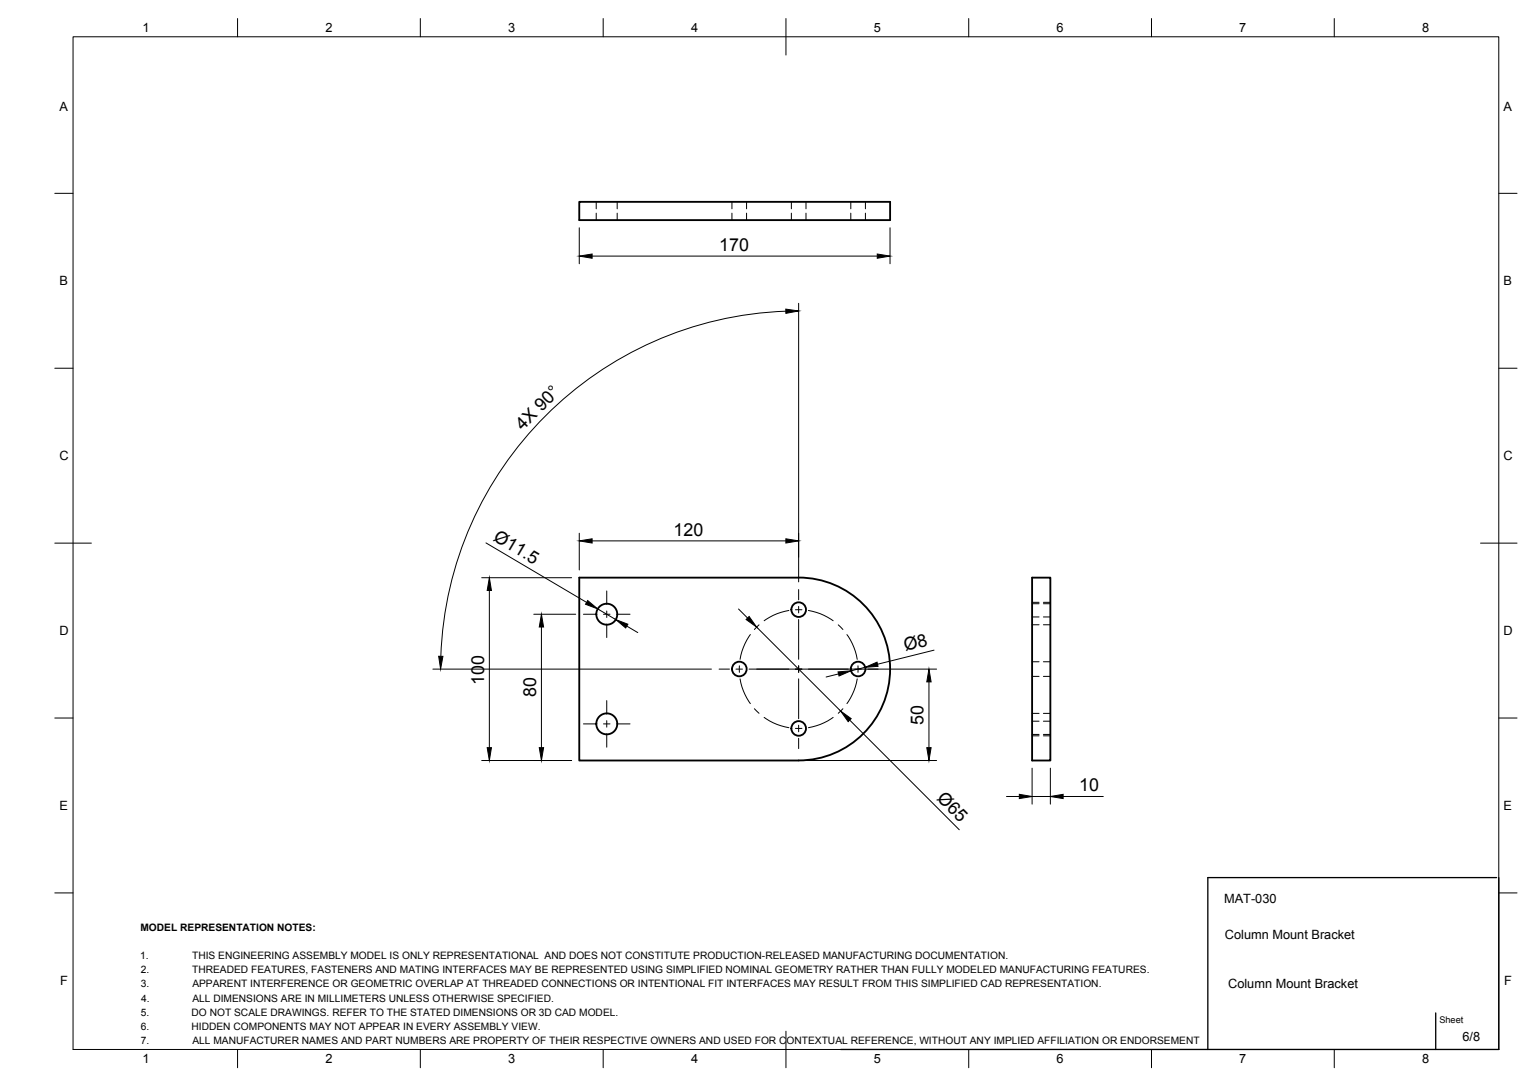
ISO-10303-21;
HEADER;
/* Generated by software containing ST-Developer
 * from STEP Tools, Inc. (www.steptools.com) 
 */

FILE_DESCRIPTION(
/* description */ ('STEP AP214'),
/* implementation_level */ '2;1');

FILE_NAME(
/* name */ 'Column Mount Bracket.step',
/* time_stamp */ '2026-11-14T06:43:04-08:00',
/* author */ (''),
/* organization */ (''),
/* preprocessor_version */ 'ST-DEVELOPER v20.2',
/* originating_system */ 'Autodesk Translation Framework v15.17.0.0',
/* authorisation */ '');

FILE_SCHEMA (('AUTOMOTIVE_DESIGN { 1 0 10303 214 3 1 1 }'));
ENDSEC;

DATA;
#10=MECHANICAL_DESIGN_GEOMETRIC_PRESENTATION_REPRESENTATION('',(#199),#5658);
#177=SHAPE_REPRESENTATION_RELATIONSHIP('SRR','None',#5707,#188);
#188=ADVANCED_BREP_SHAPE_REPRESENTATION('',(#210),#5648);
#199=STYLED_ITEM('',(#5771),#210);
#210=MANIFOLD_SOLID_BREP('Body1',#3061);
#224=CYLINDRICAL_SURFACE('',#3214,4.);
#225=CYLINDRICAL_SURFACE('',#3217,4.);
#226=CYLINDRICAL_SURFACE('',#3220,4.);
#227=CYLINDRICAL_SURFACE('',#3223,3.99999999999999);
#228=CYLINDRICAL_SURFACE('',#3226,5.75);
#229=CYLINDRICAL_SURFACE('',#3229,5.75000000000001);
#230=CYLINDRICAL_SURFACE('',#3238,50.0000000000001);
#273=FACE_BOUND('',#538,.T.);
#274=FACE_BOUND('',#539,.T.);
#275=FACE_BOUND('',#540,.T.);
#276=FACE_BOUND('',#541,.T.);
#277=FACE_BOUND('',#542,.T.);
#278=FACE_BOUND('',#543,.T.);
#279=FACE_BOUND('',#545,.T.);
#280=FACE_BOUND('',#546,.T.);
#281=FACE_BOUND('',#547,.T.);
#282=FACE_BOUND('',#548,.T.);
#283=FACE_BOUND('',#549,.T.);
#284=FACE_BOUND('',#550,.T.);
#347=FACE_OUTER_BOUND('',#531,.T.);
#348=FACE_OUTER_BOUND('',#532,.T.);
#349=FACE_OUTER_BOUND('',#533,.T.);
#350=FACE_OUTER_BOUND('',#534,.T.);
#351=FACE_OUTER_BOUND('',#535,.T.);
#352=FACE_OUTER_BOUND('',#536,.T.);
#353=FACE_OUTER_BOUND('',#537,.T.);
#354=FACE_OUTER_BOUND('',#544,.T.);
#355=FACE_OUTER_BOUND('',#551,.T.);
#356=FACE_OUTER_BOUND('',#552,.T.);
#357=FACE_OUTER_BOUND('',#553,.T.);
#358=FACE_OUTER_BOUND('',#554,.T.);
#531=EDGE_LOOP('',(#2024,#2025,#2026,#2027));
#532=EDGE_LOOP('',(#2028,#2029,#2030,#2031));
#533=EDGE_LOOP('',(#2032,#2033,#2034,#2035));
#534=EDGE_LOOP('',(#2036,#2037,#2038,#2039));
#535=EDGE_LOOP('',(#2040,#2041,#2042,#2043));
#536=EDGE_LOOP('',(#2044,#2045,#2046,#2047));
#537=EDGE_LOOP('',(#2048,#2049,#2050,#2051));
#538=EDGE_LOOP('',(#2052));
#539=EDGE_LOOP('',(#2053));
#540=EDGE_LOOP('',(#2054));
#541=EDGE_LOOP('',(#2055));
#542=EDGE_LOOP('',(#2056));
#543=EDGE_LOOP('',(#2057));
#544=EDGE_LOOP('',(#2058,#2059,#2060,#2061));
#545=EDGE_LOOP('',(#2062));
#546=EDGE_LOOP('',(#2063));
#547=EDGE_LOOP('',(#2064));
#548=EDGE_LOOP('',(#2065));
#549=EDGE_LOOP('',(#2066));
#550=EDGE_LOOP('',(#2067));
#551=EDGE_LOOP('',(#2068,#2069,#2070,#2071));
#552=EDGE_LOOP('',(#2072,#2073,#2074,#2075));
#553=EDGE_LOOP('',(#2076,#2077,#2078,#2079));
#554=EDGE_LOOP('',(#2080,#2081,#2082,#2083));
#783=LINE('',#4544,#979);
#784=LINE('',#4550,#980);
#785=LINE('',#4556,#981);
#786=LINE('',#4562,#982);
#787=LINE('',#4568,#983);
#788=LINE('',#4574,#984);
#789=LINE('',#4579,#985);
#790=LINE('',#4581,#986);
#791=LINE('',#4584,#987);
#792=LINE('',#4588,#988);
#793=LINE('',#4590,#989);
#794=LINE('',#4593,#990);
#795=LINE('',#4595,#991);
#796=LINE('',#4596,#992);
#797=LINE('',#4598,#993);
#798=LINE('',#4600,#994);
#979=VECTOR('',#3621,4.);
#980=VECTOR('',#3628,4.);
#981=VECTOR('',#3635,4.);
#982=VECTOR('',#3642,3.99999999999999);
#983=VECTOR('',#3649,5.75);
#984=VECTOR('',#3656,5.75000000000001);
#985=VECTOR('',#3661,1000.);
#986=VECTOR('',#3662,1000.);
#987=VECTOR('',#3665,1000.);
#988=VECTOR('',#3668,1000.);
#989=VECTOR('',#3669,1000.);
#990=VECTOR('',#3672,1000.);
#991=VECTOR('',#3675,1000.);
#992=VECTOR('',#3676,1000.);
#993=VECTOR('',#3679,1000.);
#994=VECTOR('',#3682,1000.);
#1167=CIRCLE('',#3215,4.);
#1168=CIRCLE('',#3216,4.);
#1169=CIRCLE('',#3218,4.);
#1170=CIRCLE('',#3219,4.);
#1171=CIRCLE('',#3221,4.00000000000001);
#1172=CIRCLE('',#3222,4.00000000000001);
#1173=CIRCLE('',#3224,3.99999999999999);
#1174=CIRCLE('',#3225,3.99999999999999);
#1175=CIRCLE('',#3227,5.75);
#1176=CIRCLE('',#3228,5.75);
#1177=CIRCLE('',#3230,5.75000000000001);
#1178=CIRCLE('',#3231,5.75000000000001);
#1179=CIRCLE('',#3233,50.0000000000001);
#1180=CIRCLE('',#3235,50.0000000000001);
#1330=VERTEX_POINT('',#4541);
#1331=VERTEX_POINT('',#4543);
#1332=VERTEX_POINT('',#4547);
#1333=VERTEX_POINT('',#4549);
#1334=VERTEX_POINT('',#4553);
#1335=VERTEX_POINT('',#4555);
#1336=VERTEX_POINT('',#4559);
#1337=VERTEX_POINT('',#4561);
#1338=VERTEX_POINT('',#4565);
#1339=VERTEX_POINT('',#4567);
#1340=VERTEX_POINT('',#4571);
#1341=VERTEX_POINT('',#4573);
#1342=VERTEX_POINT('',#4577);
#1343=VERTEX_POINT('',#4578);
#1344=VERTEX_POINT('',#4580);
#1345=VERTEX_POINT('',#4582);
#1346=VERTEX_POINT('',#4586);
#1347=VERTEX_POINT('',#4587);
#1348=VERTEX_POINT('',#4589);
#1349=VERTEX_POINT('',#4591);
#1595=EDGE_CURVE('',#1330,#1330,#1167,.T.);
#1596=EDGE_CURVE('',#1330,#1331,#783,.T.);
#1597=EDGE_CURVE('',#1331,#1331,#1168,.T.);
#1598=EDGE_CURVE('',#1332,#1332,#1169,.T.);
#1599=EDGE_CURVE('',#1332,#1333,#784,.T.);
#1600=EDGE_CURVE('',#1333,#1333,#1170,.T.);
#1601=EDGE_CURVE('',#1334,#1334,#1171,.T.);
#1602=EDGE_CURVE('',#1334,#1335,#785,.T.);
#1603=EDGE_CURVE('',#1335,#1335,#1172,.T.);
#1604=EDGE_CURVE('',#1336,#1336,#1173,.T.);
#1605=EDGE_CURVE('',#1336,#1337,#786,.T.);
#1606=EDGE_CURVE('',#1337,#1337,#1174,.T.);
#1607=EDGE_CURVE('',#1338,#1338,#1175,.T.);
#1608=EDGE_CURVE('',#1338,#1339,#787,.T.);
#1609=EDGE_CURVE('',#1339,#1339,#1176,.T.);
#1610=EDGE_CURVE('',#1340,#1340,#1177,.T.);
#1611=EDGE_CURVE('',#1340,#1341,#788,.T.);
#1612=EDGE_CURVE('',#1341,#1341,#1178,.T.);
#1613=EDGE_CURVE('',#1342,#1343,#789,.T.);
#1614=EDGE_CURVE('',#1343,#1344,#790,.T.);
#1615=EDGE_CURVE('',#1344,#1345,#1179,.T.);
#1616=EDGE_CURVE('',#1345,#1342,#791,.T.);
#1617=EDGE_CURVE('',#1346,#1347,#792,.T.);
#1618=EDGE_CURVE('',#1348,#1346,#793,.T.);
#1619=EDGE_CURVE('',#1349,#1348,#1180,.T.);
#1620=EDGE_CURVE('',#1347,#1349,#794,.T.);
#1621=EDGE_CURVE('',#1343,#1347,#795,.T.);
#1622=EDGE_CURVE('',#1342,#1346,#796,.T.);
#1623=EDGE_CURVE('',#1344,#1349,#797,.T.);
#1624=EDGE_CURVE('',#1345,#1348,#798,.T.);
#2024=ORIENTED_EDGE('',*,*,#1595,.T.);
#2025=ORIENTED_EDGE('',*,*,#1596,.T.);
#2026=ORIENTED_EDGE('',*,*,#1597,.F.);
#2027=ORIENTED_EDGE('',*,*,#1596,.F.);
#2028=ORIENTED_EDGE('',*,*,#1598,.T.);
#2029=ORIENTED_EDGE('',*,*,#1599,.T.);
#2030=ORIENTED_EDGE('',*,*,#1600,.F.);
#2031=ORIENTED_EDGE('',*,*,#1599,.F.);
#2032=ORIENTED_EDGE('',*,*,#1601,.T.);
#2033=ORIENTED_EDGE('',*,*,#1602,.T.);
#2034=ORIENTED_EDGE('',*,*,#1603,.F.);
#2035=ORIENTED_EDGE('',*,*,#1602,.F.);
#2036=ORIENTED_EDGE('',*,*,#1604,.T.);
#2037=ORIENTED_EDGE('',*,*,#1605,.T.);
#2038=ORIENTED_EDGE('',*,*,#1606,.F.);
#2039=ORIENTED_EDGE('',*,*,#1605,.F.);
#2040=ORIENTED_EDGE('',*,*,#1607,.T.);
#2041=ORIENTED_EDGE('',*,*,#1608,.T.);
#2042=ORIENTED_EDGE('',*,*,#1609,.F.);
#2043=ORIENTED_EDGE('',*,*,#1608,.F.);
#2044=ORIENTED_EDGE('',*,*,#1610,.T.);
#2045=ORIENTED_EDGE('',*,*,#1611,.T.);
#2046=ORIENTED_EDGE('',*,*,#1612,.F.);
#2047=ORIENTED_EDGE('',*,*,#1611,.F.);
#2048=ORIENTED_EDGE('',*,*,#1613,.T.);
#2049=ORIENTED_EDGE('',*,*,#1614,.T.);
#2050=ORIENTED_EDGE('',*,*,#1615,.T.);
#2051=ORIENTED_EDGE('',*,*,#1616,.T.);
#2052=ORIENTED_EDGE('',*,*,#1607,.F.);
#2053=ORIENTED_EDGE('',*,*,#1601,.F.);
#2054=ORIENTED_EDGE('',*,*,#1595,.F.);
#2055=ORIENTED_EDGE('',*,*,#1598,.F.);
#2056=ORIENTED_EDGE('',*,*,#1604,.F.);
#2057=ORIENTED_EDGE('',*,*,#1610,.F.);
#2058=ORIENTED_EDGE('',*,*,#1617,.F.);
#2059=ORIENTED_EDGE('',*,*,#1618,.F.);
#2060=ORIENTED_EDGE('',*,*,#1619,.F.);
#2061=ORIENTED_EDGE('',*,*,#1620,.F.);
#2062=ORIENTED_EDGE('',*,*,#1612,.T.);
#2063=ORIENTED_EDGE('',*,*,#1609,.T.);
#2064=ORIENTED_EDGE('',*,*,#1606,.T.);
#2065=ORIENTED_EDGE('',*,*,#1603,.T.);
#2066=ORIENTED_EDGE('',*,*,#1600,.T.);
#2067=ORIENTED_EDGE('',*,*,#1597,.T.);
#2068=ORIENTED_EDGE('',*,*,#1617,.T.);
#2069=ORIENTED_EDGE('',*,*,#1621,.F.);
#2070=ORIENTED_EDGE('',*,*,#1613,.F.);
#2071=ORIENTED_EDGE('',*,*,#1622,.T.);
#2072=ORIENTED_EDGE('',*,*,#1620,.T.);
#2073=ORIENTED_EDGE('',*,*,#1623,.F.);
#2074=ORIENTED_EDGE('',*,*,#1614,.F.);
#2075=ORIENTED_EDGE('',*,*,#1621,.T.);
#2076=ORIENTED_EDGE('',*,*,#1619,.T.);
#2077=ORIENTED_EDGE('',*,*,#1624,.F.);
#2078=ORIENTED_EDGE('',*,*,#1615,.F.);
#2079=ORIENTED_EDGE('',*,*,#1623,.T.);
#2080=ORIENTED_EDGE('',*,*,#1618,.T.);
#2081=ORIENTED_EDGE('',*,*,#1622,.F.);
#2082=ORIENTED_EDGE('',*,*,#1616,.F.);
#2083=ORIENTED_EDGE('',*,*,#1624,.T.);
#2792=PLANE('',#3232);
#2793=PLANE('',#3234);
#2794=PLANE('',#3236);
#2795=PLANE('',#3237);
#2796=PLANE('',#3239);
#2888=ADVANCED_FACE('',(#347),#224,.F.);
#2889=ADVANCED_FACE('',(#348),#225,.F.);
#2890=ADVANCED_FACE('',(#349),#226,.F.);
#2891=ADVANCED_FACE('',(#350),#227,.F.);
#2892=ADVANCED_FACE('',(#351),#228,.F.);
#2893=ADVANCED_FACE('',(#352),#229,.F.);
#2894=ADVANCED_FACE('',(#353,#273,#274,#275,#276,#277,#278),#2792,.T.);
#2895=ADVANCED_FACE('',(#354,#279,#280,#281,#282,#283,#284),#2793,.F.);
#2896=ADVANCED_FACE('',(#355),#2794,.F.);
#2897=ADVANCED_FACE('',(#356),#2795,.F.);
#2898=ADVANCED_FACE('',(#357),#230,.T.);
#2899=ADVANCED_FACE('',(#358),#2796,.F.);
#3061=CLOSED_SHELL('',(#2888,#2889,#2890,#2891,#2892,#2893,#2894,#2895,
#2896,#2897,#2898,#2899));
#3213=AXIS2_PLACEMENT_3D('',#4539,#3615,#3616);
#3214=AXIS2_PLACEMENT_3D('',#4540,#3617,#3618);
#3215=AXIS2_PLACEMENT_3D('',#4542,#3619,#3620);
#3216=AXIS2_PLACEMENT_3D('',#4545,#3622,#3623);
#3217=AXIS2_PLACEMENT_3D('',#4546,#3624,#3625);
#3218=AXIS2_PLACEMENT_3D('',#4548,#3626,#3627);
#3219=AXIS2_PLACEMENT_3D('',#4551,#3629,#3630);
#3220=AXIS2_PLACEMENT_3D('',#4552,#3631,#3632);
#3221=AXIS2_PLACEMENT_3D('',#4554,#3633,#3634);
#3222=AXIS2_PLACEMENT_3D('',#4557,#3636,#3637);
#3223=AXIS2_PLACEMENT_3D('',#4558,#3638,#3639);
#3224=AXIS2_PLACEMENT_3D('',#4560,#3640,#3641);
#3225=AXIS2_PLACEMENT_3D('',#4563,#3643,#3644);
#3226=AXIS2_PLACEMENT_3D('',#4564,#3645,#3646);
#3227=AXIS2_PLACEMENT_3D('',#4566,#3647,#3648);
#3228=AXIS2_PLACEMENT_3D('',#4569,#3650,#3651);
#3229=AXIS2_PLACEMENT_3D('',#4570,#3652,#3653);
#3230=AXIS2_PLACEMENT_3D('',#4572,#3654,#3655);
#3231=AXIS2_PLACEMENT_3D('',#4575,#3657,#3658);
#3232=AXIS2_PLACEMENT_3D('',#4576,#3659,#3660);
#3233=AXIS2_PLACEMENT_3D('',#4583,#3663,#3664);
#3234=AXIS2_PLACEMENT_3D('',#4585,#3666,#3667);
#3235=AXIS2_PLACEMENT_3D('',#4592,#3670,#3671);
#3236=AXIS2_PLACEMENT_3D('',#4594,#3673,#3674);
#3237=AXIS2_PLACEMENT_3D('',#4597,#3677,#3678);
#3238=AXIS2_PLACEMENT_3D('',#4599,#3680,#3681);
#3239=AXIS2_PLACEMENT_3D('',#4601,#3683,#3684);
#3615=DIRECTION('axis',(0.,0.,1.));
#3616=DIRECTION('refdir',(1.,0.,0.));
#3617=DIRECTION('center_axis',(0.,0.,-1.));
#3618=DIRECTION('ref_axis',(-1.,0.,0.));
#3619=DIRECTION('center_axis',(0.,0.,1.));
#3620=DIRECTION('ref_axis',(1.,0.,0.));
#3621=DIRECTION('',(0.,0.,-1.));
#3622=DIRECTION('center_axis',(0.,0.,1.));
#3623=DIRECTION('ref_axis',(1.,0.,0.));
#3624=DIRECTION('center_axis',(0.,0.,-1.));
#3625=DIRECTION('ref_axis',(-1.,0.,0.));
#3626=DIRECTION('center_axis',(0.,0.,1.));
#3627=DIRECTION('ref_axis',(1.,0.,0.));
#3628=DIRECTION('',(0.,0.,-1.));
#3629=DIRECTION('center_axis',(0.,0.,1.));
#3630=DIRECTION('ref_axis',(1.,0.,0.));
#3631=DIRECTION('center_axis',(0.,0.,-1.));
#3632=DIRECTION('ref_axis',(-1.,0.,0.));
#3633=DIRECTION('center_axis',(0.,0.,1.));
#3634=DIRECTION('ref_axis',(1.,0.,0.));
#3635=DIRECTION('',(0.,0.,-1.));
#3636=DIRECTION('center_axis',(0.,0.,1.));
#3637=DIRECTION('ref_axis',(1.,0.,0.));
#3638=DIRECTION('center_axis',(0.,0.,-1.));
#3639=DIRECTION('ref_axis',(-1.,0.,0.));
#3640=DIRECTION('center_axis',(0.,0.,1.));
#3641=DIRECTION('ref_axis',(1.,0.,0.));
#3642=DIRECTION('',(0.,0.,-1.));
#3643=DIRECTION('center_axis',(0.,0.,1.));
#3644=DIRECTION('ref_axis',(1.,0.,0.));
#3645=DIRECTION('center_axis',(0.,0.,-1.));
#3646=DIRECTION('ref_axis',(-1.,0.,0.));
#3647=DIRECTION('center_axis',(0.,0.,1.));
#3648=DIRECTION('ref_axis',(1.,0.,0.));
#3649=DIRECTION('',(0.,0.,-1.));
#3650=DIRECTION('center_axis',(0.,0.,1.));
#3651=DIRECTION('ref_axis',(1.,0.,0.));
#3652=DIRECTION('center_axis',(0.,0.,-1.));
#3653=DIRECTION('ref_axis',(-1.,0.,0.));
#3654=DIRECTION('center_axis',(0.,0.,1.));
#3655=DIRECTION('ref_axis',(1.,0.,0.));
#3656=DIRECTION('',(0.,0.,-1.));
#3657=DIRECTION('center_axis',(0.,0.,1.));
#3658=DIRECTION('ref_axis',(1.,0.,0.));
#3659=DIRECTION('center_axis',(0.,0.,1.));
#3660=DIRECTION('ref_axis',(1.,0.,0.));
#3661=DIRECTION('',(1.,0.,0.));
#3662=DIRECTION('',(7.22801448323673E-16,1.,0.));
#3663=DIRECTION('center_axis',(0.,0.,1.));
#3664=DIRECTION('ref_axis',(1.,0.,0.));
#3665=DIRECTION('',(1.15648231731788E-15,-1.,0.));
#3666=DIRECTION('center_axis',(0.,0.,1.));
#3667=DIRECTION('ref_axis',(1.,0.,0.));
#3668=DIRECTION('',(1.,0.,0.));
#3669=DIRECTION('',(1.15648231731788E-15,-1.,0.));
#3670=DIRECTION('center_axis',(0.,0.,1.));
#3671=DIRECTION('ref_axis',(1.,0.,0.));
#3672=DIRECTION('',(7.22801448323673E-16,1.,0.));
#3673=DIRECTION('center_axis',(0.,1.,0.));
#3674=DIRECTION('ref_axis',(0.,0.,1.));
#3675=DIRECTION('',(0.,0.,-1.));
#3676=DIRECTION('',(0.,0.,-1.));
#3677=DIRECTION('center_axis',(-1.,7.22801448323673E-16,0.));
#3678=DIRECTION('ref_axis',(-7.22801448323673E-16,-1.,0.));
#3679=DIRECTION('',(0.,0.,-1.));
#3680=DIRECTION('center_axis',(0.,0.,-1.));
#3681=DIRECTION('ref_axis',(-1.,0.,0.));
#3682=DIRECTION('',(0.,0.,-1.));
#3683=DIRECTION('center_axis',(1.,1.15648231731788E-15,0.));
#3684=DIRECTION('ref_axis',(-1.15648231731788E-15,1.,0.));
#4539=CARTESIAN_POINT('',(0.,0.,0.));
#4540=CARTESIAN_POINT('Origin',(-82.5,120.,10.));
#4541=CARTESIAN_POINT('',(-78.5,120.,10.));
#4542=CARTESIAN_POINT('Origin',(-82.5,120.,10.));
#4543=CARTESIAN_POINT('',(-78.5,120.,0.));
#4544=CARTESIAN_POINT('',(-78.5,120.,10.));
#4545=CARTESIAN_POINT('Origin',(-82.5,120.,0.));
#4546=CARTESIAN_POINT('Origin',(-50.,87.5,10.));
#4547=CARTESIAN_POINT('',(-46.,87.5,10.));
#4548=CARTESIAN_POINT('Origin',(-50.,87.5,10.));
#4549=CARTESIAN_POINT('',(-46.,87.5,0.));
#4550=CARTESIAN_POINT('',(-46.,87.5,10.));
#4551=CARTESIAN_POINT('Origin',(-50.,87.5,0.));
#4552=CARTESIAN_POINT('Origin',(-17.5,120.,10.));
#4553=CARTESIAN_POINT('',(-13.5,120.,10.));
#4554=CARTESIAN_POINT('Origin',(-17.5,120.,10.));
#4555=CARTESIAN_POINT('',(-13.5,120.,0.));
#4556=CARTESIAN_POINT('',(-13.5,120.,10.));
#4557=CARTESIAN_POINT('Origin',(-17.5,120.,0.));
#4558=CARTESIAN_POINT('Origin',(-50.,152.5,10.));
#4559=CARTESIAN_POINT('',(-46.,152.5,10.));
#4560=CARTESIAN_POINT('Origin',(-50.,152.5,10.));
#4561=CARTESIAN_POINT('',(-46.,152.5,0.));
#4562=CARTESIAN_POINT('',(-46.,152.5,10.));
#4563=CARTESIAN_POINT('Origin',(-50.,152.5,0.));
#4564=CARTESIAN_POINT('Origin',(-20.,15.,10.));
#4565=CARTESIAN_POINT('',(-14.25,15.,10.));
#4566=CARTESIAN_POINT('Origin',(-20.,15.,10.));
#4567=CARTESIAN_POINT('',(-14.25,15.,0.));
#4568=CARTESIAN_POINT('',(-14.25,15.,10.));
#4569=CARTESIAN_POINT('Origin',(-20.,15.,0.));
#4570=CARTESIAN_POINT('Origin',(-80.,15.,10.));
#4571=CARTESIAN_POINT('',(-74.25,15.,10.));
#4572=CARTESIAN_POINT('Origin',(-80.,15.,10.));
#4573=CARTESIAN_POINT('',(-74.25,15.,0.));
#4574=CARTESIAN_POINT('',(-74.25,15.,10.));
#4575=CARTESIAN_POINT('Origin',(-80.,15.,0.));
#4576=CARTESIAN_POINT('Origin',(-50.,120.,10.));
#4577=CARTESIAN_POINT('',(-100.,0.,10.));
#4578=CARTESIAN_POINT('',(0.,0.,10.));
#4579=CARTESIAN_POINT('',(0.,0.,10.));
#4580=CARTESIAN_POINT('',(8.67361737988404E-14,120.,10.));
#4581=CARTESIAN_POINT('',(0.,0.,10.));
#4582=CARTESIAN_POINT('',(-100.,119.999999999999,10.));
#4583=CARTESIAN_POINT('Origin',(-50.,120.,10.));
#4584=CARTESIAN_POINT('',(-100.,0.,10.));
#4585=CARTESIAN_POINT('Origin',(-50.,120.,0.));
#4586=CARTESIAN_POINT('',(-100.,0.,0.));
#4587=CARTESIAN_POINT('',(0.,0.,0.));
#4588=CARTESIAN_POINT('',(0.,0.,0.));
#4589=CARTESIAN_POINT('',(-100.,119.999999999999,0.));
#4590=CARTESIAN_POINT('',(-100.,0.,0.));
#4591=CARTESIAN_POINT('',(8.67361737988404E-14,120.,0.));
#4592=CARTESIAN_POINT('Origin',(-50.,120.,0.));
#4593=CARTESIAN_POINT('',(0.,0.,0.));
#4594=CARTESIAN_POINT('Origin',(0.,0.,10.));
#4595=CARTESIAN_POINT('',(0.,0.,10.));
#4596=CARTESIAN_POINT('',(-100.,0.,10.));
#4597=CARTESIAN_POINT('Origin',(0.,0.,10.));
#4598=CARTESIAN_POINT('',(8.67361737988404E-14,120.,10.));
#4599=CARTESIAN_POINT('Origin',(-50.,120.,10.));
#4600=CARTESIAN_POINT('',(-100.,119.999999999999,10.));
#4601=CARTESIAN_POINT('Origin',(-100.,0.,10.));
#5635=UNCERTAINTY_MEASURE_WITH_UNIT(LENGTH_MEASURE(0.01),#5659,
'DISTANCE_ACCURACY_VALUE',
'Maximum model space distance between geometric entities at asserted c
onnectivities');
#5645=UNCERTAINTY_MEASURE_WITH_UNIT(LENGTH_MEASURE(0.01),#5659,
'DISTANCE_ACCURACY_VALUE',
'Maximum model space distance between geometric entities at asserted c
onnectivities');
#5648=(
GEOMETRIC_REPRESENTATION_CONTEXT(3)
GLOBAL_UNCERTAINTY_ASSIGNED_CONTEXT((#5635))
GLOBAL_UNIT_ASSIGNED_CONTEXT((#5659,#5661,#5662))
REPRESENTATION_CONTEXT('','3D')
);
#5658=(
GEOMETRIC_REPRESENTATION_CONTEXT(3)
GLOBAL_UNCERTAINTY_ASSIGNED_CONTEXT((#5645))
GLOBAL_UNIT_ASSIGNED_CONTEXT((#5659,#5661,#5662))
REPRESENTATION_CONTEXT('','3D')
);
#5659=(
LENGTH_UNIT()
NAMED_UNIT(*)
SI_UNIT(.MILLI.,.METRE.)
);
#5661=(
NAMED_UNIT(*)
PLANE_ANGLE_UNIT()
SI_UNIT($,.RADIAN.)
);
#5662=(
NAMED_UNIT(*)
SI_UNIT($,.STERADIAN.)
SOLID_ANGLE_UNIT()
);
#5665=SHAPE_DEFINITION_REPRESENTATION(#5677,#5707);
#5677=PRODUCT_DEFINITION_SHAPE('',$,#5720);
#5707=SHAPE_REPRESENTATION('',(#3213),#5648);
#5717=PRODUCT_DEFINITION_CONTEXT('part definition',#5755,'design');
#5720=PRODUCT_DEFINITION('Column Mount Bracket','Column Mount Bracket',
#5732,#5717);
#5732=PRODUCT_DEFINITION_FORMATION('',$,#5759);
#5755=APPLICATION_CONTEXT(
'Core Data for Automotive Mechanical Design Process');
#5756=PRODUCT_CONTEXT('part definition',#5755,'mechanical');
#5759=PRODUCT('Column Mount Bracket','Column Mount Bracket',$,(#5756));
#5771=PRESENTATION_STYLE_ASSIGNMENT((#5776));
#5776=SURFACE_STYLE_USAGE(.BOTH.,#5781);
#5781=SURFACE_SIDE_STYLE('',(#5786));
#5786=SURFACE_STYLE_FILL_AREA(#5791);
#5791=FILL_AREA_STYLE('Opaque(20,51,87)',(#5796));
#5796=FILL_AREA_STYLE_COLOUR('Opaque(20,51,87)',#5801);
#5801=COLOUR_RGB('Opaque(20,51,87)',0.0784313725490196,0.2,0.341176470588235);
ENDSEC;
END-ISO-10303-21;
